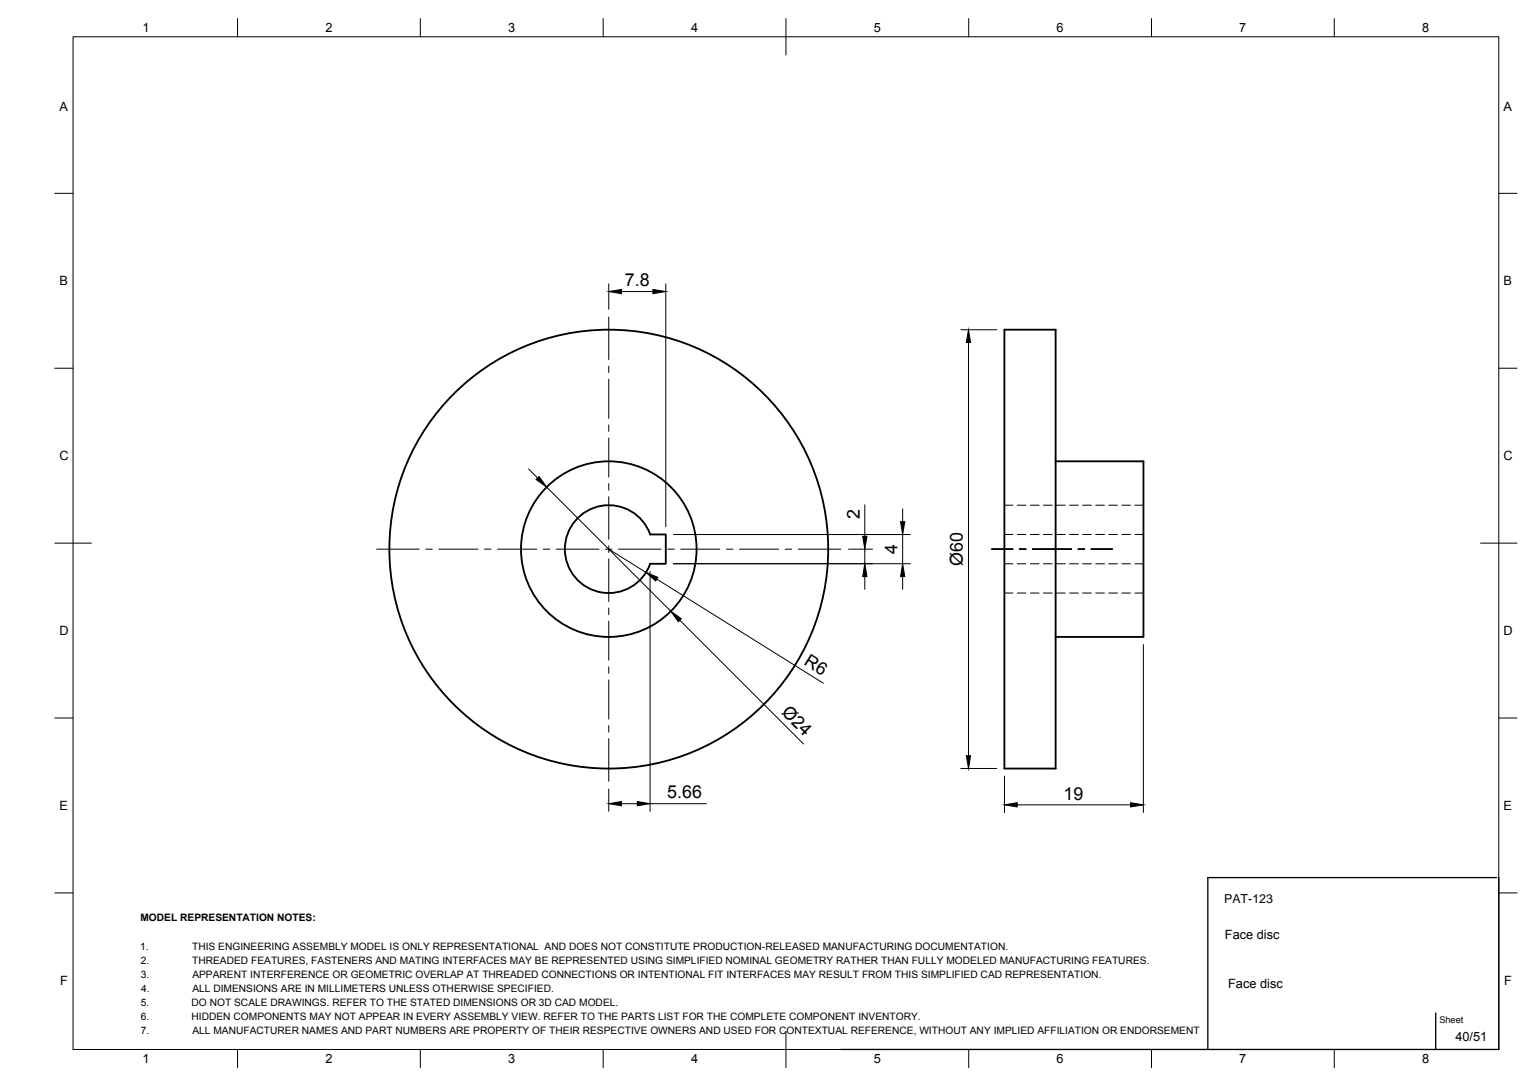
ISO-10303-21;
HEADER;
/* Generated by software containing ST-Developer
 * from STEP Tools, Inc. (www.steptools.com) 
 */

FILE_DESCRIPTION(
/* description */ ('Worm-less right-angle friction wheel drive'),
/* implementation_level */ '2;1');

FILE_NAME(
/* name */ 'Face disc.step',
/* time_stamp */ '2026-10-28T03:22:36-07:00',
/* author */ (''),
/* organization */ (''),
/* preprocessor_version */ 'ST-DEVELOPER v20.2',
/* originating_system */ 'Autodesk Translation Framework v15.17.0.0',
/* authorisation */ '');

FILE_SCHEMA (('AUTOMOTIVE_DESIGN { 1 0 10303 214 3 1 1 }'));
ENDSEC;

DATA;
#10=MECHANICAL_DESIGN_GEOMETRIC_PRESENTATION_REPRESENTATION('',(#653),#17046);
#552=SHAPE_REPRESENTATION_RELATIONSHIP('SRR','None',#17297,#599);
#599=ADVANCED_BREP_SHAPE_REPRESENTATION('',(#704),#17033);
#653=STYLED_ITEM('',(#17605),#704);
#704=MANIFOLD_SOLID_BREP('Body1',#8211);
#929=FACE_BOUND('',#2260,.T.);
#930=FACE_BOUND('',#2263,.T.);
#931=FACE_BOUND('',#2267,.T.);
#1141=PLANE('',#9506);
#1142=PLANE('',#9507);
#1143=PLANE('',#9508);
#1144=PLANE('',#9509);
#1145=PLANE('',#9514);
#1146=PLANE('',#9520);
#1576=FACE_OUTER_BOUND('',#2256,.T.);
#1577=FACE_OUTER_BOUND('',#2257,.T.);
#1578=FACE_OUTER_BOUND('',#2258,.T.);
#1579=FACE_OUTER_BOUND('',#2259,.T.);
#1580=FACE_OUTER_BOUND('',#2261,.T.);
#1581=FACE_OUTER_BOUND('',#2262,.T.);
#1582=FACE_OUTER_BOUND('',#2264,.T.);
#1583=FACE_OUTER_BOUND('',#2265,.T.);
#1584=FACE_OUTER_BOUND('',#2266,.T.);
#2256=EDGE_LOOP('',(#7130,#7131,#7132,#7133));
#2257=EDGE_LOOP('',(#7134,#7135,#7136,#7137));
#2258=EDGE_LOOP('',(#7138,#7139,#7140,#7141));
#2259=EDGE_LOOP('',(#7142));
#2260=EDGE_LOOP('',(#7143,#7144,#7145,#7146));
#2261=EDGE_LOOP('',(#7147,#7148,#7149,#7150));
#2262=EDGE_LOOP('',(#7151));
#2263=EDGE_LOOP('',(#7152));
#2264=EDGE_LOOP('',(#7153,#7154,#7155,#7156));
#2265=EDGE_LOOP('',(#7157,#7158,#7159,#7160));
#2266=EDGE_LOOP('',(#7161));
#2267=EDGE_LOOP('',(#7162,#7163,#7164,#7165));
#2790=LINE('',#16295,#3330);
#2791=LINE('',#16297,#3331);
#2792=LINE('',#16299,#3332);
#2793=LINE('',#16300,#3333);
#2794=LINE('',#16303,#3334);
#2795=LINE('',#16305,#3335);
#2796=LINE('',#16306,#3336);
#2797=LINE('',#16309,#3337);
#2798=LINE('',#16311,#3338);
#2799=LINE('',#16312,#3339);
#2800=LINE('',#16325,#3340);
#2801=LINE('',#16328,#3341);
#3330=VECTOR('',#11716,1.);
#3331=VECTOR('',#11717,1.);
#3332=VECTOR('',#11718,1.);
#3333=VECTOR('',#11719,1.);
#3334=VECTOR('',#11722,1.);
#3335=VECTOR('',#11723,1.);
#3336=VECTOR('',#11724,1.);
#3337=VECTOR('',#11727,1.);
#3338=VECTOR('',#11728,1.);
#3339=VECTOR('',#11729,1.);
#3340=VECTOR('',#11748,3.);
#3341=VECTOR('',#11751,1.2);
#3810=CIRCLE('',#9510,3.);
#3811=CIRCLE('',#9511,0.6);
#3812=CIRCLE('',#9513,0.6);
#3813=CIRCLE('',#9515,3.);
#3814=CIRCLE('',#9516,1.2);
#3815=CIRCLE('',#9519,1.2);
#4405=VERTEX_POINT('',#16293);
#4406=VERTEX_POINT('',#16294);
#4407=VERTEX_POINT('',#16296);
#4408=VERTEX_POINT('',#16298);
#4409=VERTEX_POINT('',#16302);
#4410=VERTEX_POINT('',#16304);
#4411=VERTEX_POINT('',#16308);
#4412=VERTEX_POINT('',#16310);
#4413=VERTEX_POINT('',#16314);
#4414=VERTEX_POINT('',#16320);
#4415=VERTEX_POINT('',#16322);
#4416=VERTEX_POINT('',#16327);
#5334=EDGE_CURVE('',#4405,#4406,#2790,.T.);
#5335=EDGE_CURVE('',#4405,#4407,#2791,.T.);
#5336=EDGE_CURVE('',#4408,#4407,#2792,.T.);
#5337=EDGE_CURVE('',#4406,#4408,#2793,.T.);
#5338=EDGE_CURVE('',#4409,#4405,#2794,.T.);
#5339=EDGE_CURVE('',#4409,#4410,#2795,.T.);
#5340=EDGE_CURVE('',#4407,#4410,#2796,.T.);
#5341=EDGE_CURVE('',#4411,#4409,#2797,.T.);
#5342=EDGE_CURVE('',#4412,#4411,#2798,.T.);
#5343=EDGE_CURVE('',#4410,#4412,#2799,.T.);
#5344=EDGE_CURVE('',#4413,#4413,#3810,.T.);
#5345=EDGE_CURVE('',#4412,#4408,#3811,.T.);
#5346=EDGE_CURVE('',#4411,#4406,#3812,.T.);
#5347=EDGE_CURVE('',#4414,#4414,#3813,.T.);
#5348=EDGE_CURVE('',#4415,#4415,#3814,.T.);
#5349=EDGE_CURVE('',#4413,#4414,#2800,.T.);
#5350=EDGE_CURVE('',#4415,#4416,#2801,.T.);
#5351=EDGE_CURVE('',#4416,#4416,#3815,.T.);
#7130=ORIENTED_EDGE('',*,*,#5334,.F.);
#7131=ORIENTED_EDGE('',*,*,#5335,.T.);
#7132=ORIENTED_EDGE('',*,*,#5336,.F.);
#7133=ORIENTED_EDGE('',*,*,#5337,.F.);
#7134=ORIENTED_EDGE('',*,*,#5338,.F.);
#7135=ORIENTED_EDGE('',*,*,#5339,.T.);
#7136=ORIENTED_EDGE('',*,*,#5340,.F.);
#7137=ORIENTED_EDGE('',*,*,#5335,.F.);
#7138=ORIENTED_EDGE('',*,*,#5341,.F.);
#7139=ORIENTED_EDGE('',*,*,#5342,.F.);
#7140=ORIENTED_EDGE('',*,*,#5343,.F.);
#7141=ORIENTED_EDGE('',*,*,#5339,.F.);
#7142=ORIENTED_EDGE('',*,*,#5344,.T.);
#7143=ORIENTED_EDGE('',*,*,#5336,.T.);
#7144=ORIENTED_EDGE('',*,*,#5340,.T.);
#7145=ORIENTED_EDGE('',*,*,#5343,.T.);
#7146=ORIENTED_EDGE('',*,*,#5345,.T.);
#7147=ORIENTED_EDGE('',*,*,#5337,.T.);
#7148=ORIENTED_EDGE('',*,*,#5345,.F.);
#7149=ORIENTED_EDGE('',*,*,#5342,.T.);
#7150=ORIENTED_EDGE('',*,*,#5346,.T.);
#7151=ORIENTED_EDGE('',*,*,#5347,.F.);
#7152=ORIENTED_EDGE('',*,*,#5348,.F.);
#7153=ORIENTED_EDGE('',*,*,#5344,.F.);
#7154=ORIENTED_EDGE('',*,*,#5349,.T.);
#7155=ORIENTED_EDGE('',*,*,#5347,.T.);
#7156=ORIENTED_EDGE('',*,*,#5349,.F.);
#7157=ORIENTED_EDGE('',*,*,#5348,.T.);
#7158=ORIENTED_EDGE('',*,*,#5350,.T.);
#7159=ORIENTED_EDGE('',*,*,#5351,.T.);
#7160=ORIENTED_EDGE('',*,*,#5350,.F.);
#7161=ORIENTED_EDGE('',*,*,#5351,.F.);
#7162=ORIENTED_EDGE('',*,*,#5334,.T.);
#7163=ORIENTED_EDGE('',*,*,#5346,.F.);
#7164=ORIENTED_EDGE('',*,*,#5341,.T.);
#7165=ORIENTED_EDGE('',*,*,#5338,.T.);
#7674=CYLINDRICAL_SURFACE('',#9512,0.6);
#7675=CYLINDRICAL_SURFACE('',#9517,3.);
#7676=CYLINDRICAL_SURFACE('',#9518,1.2);
#8068=ADVANCED_FACE('',(#1576),#1141,.F.);
#8069=ADVANCED_FACE('',(#1577),#1142,.F.);
#8070=ADVANCED_FACE('',(#1578),#1143,.F.);
#8071=ADVANCED_FACE('',(#1579,#929),#1144,.T.);
#8072=ADVANCED_FACE('',(#1580),#7674,.F.);
#8073=ADVANCED_FACE('',(#1581,#930),#1145,.F.);
#8074=ADVANCED_FACE('',(#1582),#7675,.T.);
#8075=ADVANCED_FACE('',(#1583),#7676,.T.);
#8076=ADVANCED_FACE('',(#1584,#931),#1146,.F.);
#8211=CLOSED_SHELL('',(#8068,#8069,#8070,#8071,#8072,#8073,#8074,#8075,
#8076));
#9505=AXIS2_PLACEMENT_3D('',#16291,#11712,#11713);
#9506=AXIS2_PLACEMENT_3D('',#16292,#11714,#11715);
#9507=AXIS2_PLACEMENT_3D('',#16301,#11720,#11721);
#9508=AXIS2_PLACEMENT_3D('',#16307,#11725,#11726);
#9509=AXIS2_PLACEMENT_3D('',#16313,#11730,#11731);
#9510=AXIS2_PLACEMENT_3D('',#16315,#11732,#11733);
#9511=AXIS2_PLACEMENT_3D('',#16316,#11734,#11735);
#9512=AXIS2_PLACEMENT_3D('',#16317,#11736,#11737);
#9513=AXIS2_PLACEMENT_3D('',#16318,#11738,#11739);
#9514=AXIS2_PLACEMENT_3D('',#16319,#11740,#11741);
#9515=AXIS2_PLACEMENT_3D('',#16321,#11742,#11743);
#9516=AXIS2_PLACEMENT_3D('',#16323,#11744,#11745);
#9517=AXIS2_PLACEMENT_3D('',#16324,#11746,#11747);
#9518=AXIS2_PLACEMENT_3D('',#16326,#11749,#11750);
#9519=AXIS2_PLACEMENT_3D('',#16329,#11752,#11753);
#9520=AXIS2_PLACEMENT_3D('',#16330,#11754,#11755);
#11712=DIRECTION('axis',(0.,0.,1.));
#11713=DIRECTION('refdir',(1.,0.,0.));
#11714=DIRECTION('center_axis',(-1.,0.,0.));
#11715=DIRECTION('ref_axis',(0.,0.,1.));
#11716=DIRECTION('',(0.,0.,1.));
#11717=DIRECTION('',(0.,1.,0.));
#11718=DIRECTION('',(0.,0.,-1.));
#11719=DIRECTION('',(0.,1.,0.));
#11720=DIRECTION('center_axis',(0.,0.,-1.));
#11721=DIRECTION('ref_axis',(-1.,0.,0.));
#11722=DIRECTION('',(-1.,0.,0.));
#11723=DIRECTION('',(0.,1.,0.));
#11724=DIRECTION('',(1.,0.,0.));
#11725=DIRECTION('center_axis',(1.,0.,0.));
#11726=DIRECTION('ref_axis',(0.,0.,-1.));
#11727=DIRECTION('',(0.,0.,-1.));
#11728=DIRECTION('',(0.,-1.,0.));
#11729=DIRECTION('',(0.,0.,1.));
#11730=DIRECTION('center_axis',(0.,1.,0.));
#11731=DIRECTION('ref_axis',(1.,0.,0.));
#11732=DIRECTION('center_axis',(0.,1.,0.));
#11733=DIRECTION('ref_axis',(1.,0.,0.));
#11734=DIRECTION('center_axis',(0.,-1.,0.));
#11735=DIRECTION('ref_axis',(1.,0.,0.));
#11736=DIRECTION('center_axis',(0.,1.,0.));
#11737=DIRECTION('ref_axis',(-1.83697019872103E-16,0.,1.));
#11738=DIRECTION('center_axis',(0.,-1.,0.));
#11739=DIRECTION('ref_axis',(1.,0.,0.));
#11740=DIRECTION('center_axis',(0.,1.,0.));
#11741=DIRECTION('ref_axis',(1.,0.,0.));
#11742=DIRECTION('center_axis',(0.,1.,0.));
#11743=DIRECTION('ref_axis',(1.,0.,0.));
#11744=DIRECTION('center_axis',(0.,-1.,0.));
#11745=DIRECTION('ref_axis',(1.,0.,0.));
#11746=DIRECTION('center_axis',(0.,1.,0.));
#11747=DIRECTION('ref_axis',(1.,0.,0.));
#11748=DIRECTION('',(0.,-1.,0.));
#11749=DIRECTION('center_axis',(0.,1.,0.));
#11750=DIRECTION('ref_axis',(1.,0.,0.));
#11751=DIRECTION('',(0.,-1.,0.));
#11752=DIRECTION('center_axis',(0.,1.,0.));
#11753=DIRECTION('ref_axis',(1.,0.,0.));
#11754=DIRECTION('center_axis',(0.,1.,0.));
#11755=DIRECTION('ref_axis',(1.,0.,0.));
#16291=CARTESIAN_POINT('',(0.,0.,0.));
#16292=CARTESIAN_POINT('Origin',(-0.2,-2.1,6.22));
#16293=CARTESIAN_POINT('',(-0.2,-2.,6.22));
#16294=CARTESIAN_POINT('',(-0.2,-2.,6.43431457505076));
#16295=CARTESIAN_POINT('',(-0.2,-2.,6.61));
#16296=CARTESIAN_POINT('',(-0.2,-0.1,6.22));
#16297=CARTESIAN_POINT('',(-0.2,-2.1,6.22));
#16298=CARTESIAN_POINT('',(-0.2,-0.1,6.43431457505076));
#16299=CARTESIAN_POINT('',(-0.2,-0.0999999999999999,6.61));
#16300=CARTESIAN_POINT('',(-0.2,-2.,6.43431457505076));
#16301=CARTESIAN_POINT('Origin',(0.2,-2.1,6.22));
#16302=CARTESIAN_POINT('',(0.2,-2.,6.22));
#16303=CARTESIAN_POINT('',(0.1,-2.,6.22));
#16304=CARTESIAN_POINT('',(0.2,-0.1,6.22));
#16305=CARTESIAN_POINT('',(0.2,-2.1,6.22));
#16306=CARTESIAN_POINT('',(0.1,-0.0999999999999999,6.22));
#16307=CARTESIAN_POINT('Origin',(0.2,-2.1,7.));
#16308=CARTESIAN_POINT('',(0.2,-2.,6.43431457505076));
#16309=CARTESIAN_POINT('',(0.2,-2.,7.));
#16310=CARTESIAN_POINT('',(0.2,-0.1,6.43431457505076));
#16311=CARTESIAN_POINT('',(0.2,-2.,6.43431457505076));
#16312=CARTESIAN_POINT('',(0.2,-0.0999999999999999,7.));
#16313=CARTESIAN_POINT('Origin',(0.,-0.0999999999999999,7.));
#16314=CARTESIAN_POINT('',(-3.,-0.1,7.));
#16315=CARTESIAN_POINT('Origin',(0.,-0.1,7.));
#16316=CARTESIAN_POINT('Origin',(0.,-0.0999999999999999,7.));
#16317=CARTESIAN_POINT('Origin',(0.,-2.,7.));
#16318=CARTESIAN_POINT('Origin',(0.,-2.,7.));
#16319=CARTESIAN_POINT('Origin',(0.,-0.8,7.));
#16320=CARTESIAN_POINT('',(-3.,-0.8,7.));
#16321=CARTESIAN_POINT('Origin',(0.,-0.8,7.));
#16322=CARTESIAN_POINT('',(-1.2,-0.8,7.));
#16323=CARTESIAN_POINT('Origin',(0.,-0.8,7.));
#16324=CARTESIAN_POINT('Origin',(0.,-0.8,7.));
#16325=CARTESIAN_POINT('',(-3.,-0.8,7.));
#16326=CARTESIAN_POINT('Origin',(0.,-2.,7.));
#16327=CARTESIAN_POINT('',(-1.2,-2.,7.));
#16328=CARTESIAN_POINT('',(-1.2,-2.,7.));
#16329=CARTESIAN_POINT('Origin',(0.,-2.,7.));
#16330=CARTESIAN_POINT('Origin',(0.,-2.,7.));
#16980=UNCERTAINTY_MEASURE_WITH_UNIT(LENGTH_MEASURE(0.001),#17047,
'DISTANCE_ACCURACY_VALUE',
'Maximum model space distance between geometric entities at asserted c
onnectivities');
#16993=UNCERTAINTY_MEASURE_WITH_UNIT(LENGTH_MEASURE(0.001),#17047,
'DISTANCE_ACCURACY_VALUE',
'Maximum model space distance between geometric entities at asserted c
onnectivities');
#17033=(
GEOMETRIC_REPRESENTATION_CONTEXT(3)
GLOBAL_UNCERTAINTY_ASSIGNED_CONTEXT((#16980))
GLOBAL_UNIT_ASSIGNED_CONTEXT((#17047,#17049,#17050))
REPRESENTATION_CONTEXT('','3D')
);
#17046=(
GEOMETRIC_REPRESENTATION_CONTEXT(3)
GLOBAL_UNCERTAINTY_ASSIGNED_CONTEXT((#16993))
GLOBAL_UNIT_ASSIGNED_CONTEXT((#17047,#17049,#17050))
REPRESENTATION_CONTEXT('','3D')
);
#17047=(
LENGTH_UNIT()
NAMED_UNIT(*)
SI_UNIT(.CENTI.,.METRE.)
);
#17049=(
NAMED_UNIT(*)
PLANE_ANGLE_UNIT()
SI_UNIT($,.RADIAN.)
);
#17050=(
NAMED_UNIT(*)
SI_UNIT($,.STERADIAN.)
SOLID_ANGLE_UNIT()
);
#17090=SHAPE_DEFINITION_REPRESENTATION(#17147,#17297);
#17147=PRODUCT_DEFINITION_SHAPE('',$,#17350);
#17297=SHAPE_REPRESENTATION('',(#9505),#17033);
#17310=PRODUCT_DEFINITION_CONTEXT('part definition',#17468,'design');
#17350=PRODUCT_DEFINITION('Face disc','Face disc',#17402,#17310);
#17402=PRODUCT_DEFINITION_FORMATION('',$,#17509);
#17468=APPLICATION_CONTEXT(
'Core Data for Automotive Mechanical Design Process');
#17469=PRODUCT_CONTEXT('part definition',#17468,'mechanical');
#17509=PRODUCT('Face disc','Face disc','Face disc',(#17469));
#17599=COLOUR_RGB('Off White',0.89,0.88,0.83);
#17600=FILL_AREA_STYLE_COLOUR('',#17599);
#17601=FILL_AREA_STYLE('',(#17600));
#17602=SURFACE_STYLE_FILL_AREA(#17601);
#17603=SURFACE_SIDE_STYLE('',(#17602));
#17604=SURFACE_STYLE_USAGE(.BOTH.,#17603);
#17605=PRESENTATION_STYLE_ASSIGNMENT((#17604));
ENDSEC;
END-ISO-10303-21;
